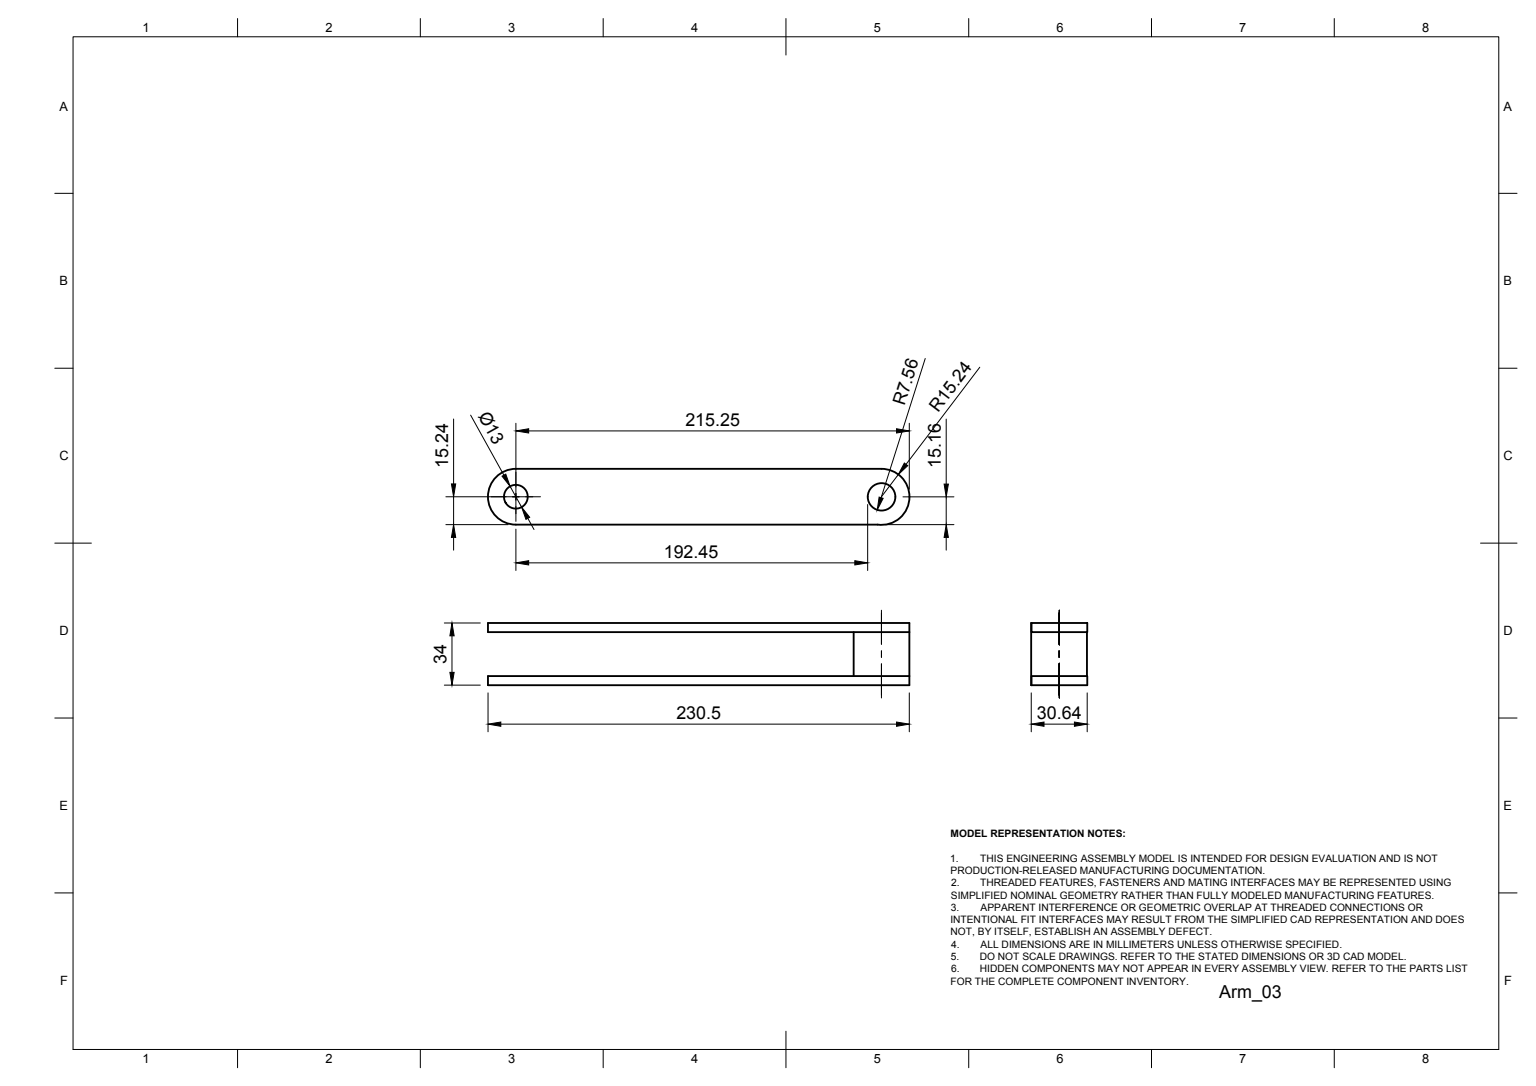
ISO-10303-21;
HEADER;
/* Generated by software containing ST-Developer
 * from STEP Tools, Inc. (www.steptools.com) 
 */

FILE_DESCRIPTION(
/* description */ (''),
/* implementation_level */ '2;1');

FILE_NAME(
/* name */ 'Arm_03.step',
/* time_stamp */ '2026-10-06T13:41:14-07:00',
/* author */ (''),
/* organization */ (''),
/* preprocessor_version */ 'ST-DEVELOPER v20.2',
/* originating_system */ 'Autodesk Translation Framework v15.15.0.0',
/* authorisation */ '');

FILE_SCHEMA (('AUTOMOTIVE_DESIGN { 1 0 10303 214 3 1 1 }'));
ENDSEC;

DATA;
#10=MECHANICAL_DESIGN_GEOMETRIC_PRESENTATION_REPRESENTATION('',(#1965),#279266);
#1947=SHAPE_REPRESENTATION_RELATIONSHIP('SRR','None',#279306,#1956);
#1956=ADVANCED_BREP_SHAPE_REPRESENTATION('',(#1974),#279262);
#1965=STYLED_ITEM('',(#279355),#1974);
#1974=MANIFOLD_SOLID_BREP('Body1',#14943);
#2002=FACE_BOUND('',#2985,.T.);
#2003=FACE_BOUND('',#2992,.T.);
#2004=FACE_BOUND('',#2993,.T.);
#2005=FACE_BOUND('',#2996,.T.);
#2006=FACE_BOUND('',#2997,.T.);
#2007=FACE_BOUND('',#2999,.T.);
#2071=PLANE('',#15521);
#2072=PLANE('',#15522);
#2073=PLANE('',#15526);
#2074=PLANE('',#15529);
#2075=PLANE('',#15534);
#2076=PLANE('',#15538);
#2077=PLANE('',#15542);
#2078=PLANE('',#15547);
#2079=PLANE('',#15549);
#2080=PLANE('',#15551);
#2486=FACE_OUTER_BOUND('',#2980,.T.);
#2487=FACE_OUTER_BOUND('',#2981,.T.);
#2488=FACE_OUTER_BOUND('',#2982,.T.);
#2489=FACE_OUTER_BOUND('',#2983,.T.);
#2490=FACE_OUTER_BOUND('',#2984,.T.);
#2491=FACE_OUTER_BOUND('',#2986,.T.);
#2492=FACE_OUTER_BOUND('',#2987,.T.);
#2493=FACE_OUTER_BOUND('',#2988,.T.);
#2494=FACE_OUTER_BOUND('',#2989,.T.);
#2495=FACE_OUTER_BOUND('',#2990,.T.);
#2496=FACE_OUTER_BOUND('',#2991,.T.);
#2497=FACE_OUTER_BOUND('',#2994,.T.);
#2498=FACE_OUTER_BOUND('',#2995,.T.);
#2499=FACE_OUTER_BOUND('',#2998,.T.);
#2500=FACE_OUTER_BOUND('',#3000,.T.);
#2501=FACE_OUTER_BOUND('',#3001,.T.);
#2502=FACE_OUTER_BOUND('',#3002,.T.);
#2503=FACE_OUTER_BOUND('',#3003,.T.);
#2504=FACE_OUTER_BOUND('',#3004,.T.);
#2505=FACE_OUTER_BOUND('',#3005,.T.);
#2980=EDGE_LOOP('',(#13442,#13443,#13444,#13445,#13446,#13447,#13448,#13449,
#13450,#13451,#13452,#13453));
#2981=EDGE_LOOP('',(#13454,#13455,#13456,#13457,#13458,#13459,#13460,#13461,
#13462,#13463,#13464,#13465));
#2982=EDGE_LOOP('',(#13466,#13467,#13468,#13469));
#2983=EDGE_LOOP('',(#13470,#13471,#13472,#13473));
#2984=EDGE_LOOP('',(#13474,#13475,#13476,#13477,#13478,#13479));
#2985=EDGE_LOOP('',(#13480));
#2986=EDGE_LOOP('',(#13481,#13482));
#2987=EDGE_LOOP('',(#13483,#13484,#13485,#13486));
#2988=EDGE_LOOP('',(#13487,#13488,#13489,#13490));
#2989=EDGE_LOOP('',(#13491,#13492,#13493,#13494));
#2990=EDGE_LOOP('',(#13495,#13496,#13497,#13498));
#2991=EDGE_LOOP('',(#13499,#13500,#13501,#13502,#13503));
#2992=EDGE_LOOP('',(#13504));
#2993=EDGE_LOOP('',(#13505,#13506,#13507));
#2994=EDGE_LOOP('',(#13508,#13509,#13510,#13511));
#2995=EDGE_LOOP('',(#13512,#13513,#13514,#13515,#13516));
#2996=EDGE_LOOP('',(#13517));
#2997=EDGE_LOOP('',(#13518,#13519,#13520));
#2998=EDGE_LOOP('',(#13521,#13522,#13523,#13524,#13525,#13526));
#2999=EDGE_LOOP('',(#13527));
#3000=EDGE_LOOP('',(#13528,#13529,#13530,#13531));
#3001=EDGE_LOOP('',(#13532,#13533,#13534,#13535));
#3002=EDGE_LOOP('',(#13536,#13537,#13538,#13539));
#3003=EDGE_LOOP('',(#13540,#13541,#13542,#13543));
#3004=EDGE_LOOP('',(#13544,#13545,#13546,#13547));
#3005=EDGE_LOOP('',(#13548,#13549));
#3499=LINE('',#240528,#4027);
#3500=LINE('',#240532,#4028);
#3501=LINE('',#240536,#4029);
#3502=LINE('',#240541,#4030);
#3503=LINE('',#240544,#4031);
#3504=LINE('',#240550,#4032);
#3505=LINE('',#240554,#4033);
#3506=LINE('',#240557,#4034);
#3507=LINE('',#240561,#4035);
#3508=LINE('',#240565,#4036);
#3509=LINE('',#240572,#4037);
#3510=LINE('',#240574,#4038);
#3511=LINE('',#240575,#4039);
#3512=LINE('',#240580,#4040);
#3513=LINE('',#240587,#4041);
#3514=LINE('',#240592,#4042);
#3515=LINE('',#240593,#4043);
#3516=LINE('',#240594,#4044);
#3517=LINE('',#240607,#4045);
#3518=LINE('',#240610,#4046);
#3519=LINE('',#240615,#4047);
#3520=LINE('',#240619,#4048);
#3521=LINE('',#240624,#4049);
#3522=LINE('',#240626,#4050);
#3523=LINE('',#240627,#4051);
#3524=LINE('',#240629,#4052);
#4027=VECTOR('',#16995,7.55784864301595);
#4028=VECTOR('',#16998,10.);
#4029=VECTOR('',#17001,10.);
#4030=VECTOR('',#17006,10.);
#4031=VECTOR('',#17009,10.);
#4032=VECTOR('',#17014,10.);
#4033=VECTOR('',#17017,10.);
#4034=VECTOR('',#17020,15.2420394990918);
#4035=VECTOR('',#17023,10.);
#4036=VECTOR('',#17026,10.);
#4037=VECTOR('',#17037,10.);
#4038=VECTOR('',#17038,10.);
#4039=VECTOR('',#17039,10.);
#4040=VECTOR('',#17044,10.);
#4041=VECTOR('',#17053,6.50110764916953);
#4042=VECTOR('',#17058,10.);
#4043=VECTOR('',#17059,10.);
#4044=VECTOR('',#17060,10.);
#4045=VECTOR('',#17081,10.);
#4046=VECTOR('',#17084,10.);
#4047=VECTOR('',#17089,10.);
#4048=VECTOR('',#17092,10.);
#4049=VECTOR('',#17099,6.50110764916953);
#4050=VECTOR('',#17102,10.);
#4051=VECTOR('',#17103,10.);
#4052=VECTOR('',#17106,10.);
#4232=CIRCLE('',#15505,7.55784864301595);
#4233=CIRCLE('',#15506,7.55784864301595);
#4234=CIRCLE('',#15507,7.55784864301595);
#4235=CIRCLE('',#15508,7.55784864301595);
#4236=CIRCLE('',#15509,7.55784864301595);
#4237=CIRCLE('',#15510,7.55784864301595);
#4238=CIRCLE('',#15512,15.2420394990918);
#4239=CIRCLE('',#15513,15.2420394990918);
#4240=CIRCLE('',#15514,15.2420394990918);
#4241=CIRCLE('',#15515,15.2420394990918);
#4242=CIRCLE('',#15516,15.2420394990918);
#4243=CIRCLE('',#15517,15.2420394990918);
#4244=CIRCLE('',#15519,7.55784864301595);
#4245=CIRCLE('',#15520,7.55784864301595);
#4246=CIRCLE('',#15523,15.2420394990918);
#4247=CIRCLE('',#15524,15.2420394990918);
#4248=CIRCLE('',#15525,6.50110764916953);
#4249=CIRCLE('',#15528,6.50110764916953);
#4250=CIRCLE('',#15531,15.2420394990918);
#4251=CIRCLE('',#15533,15.2420394990918);
#4252=CIRCLE('',#15536,7.55784864301595);
#4253=CIRCLE('',#15537,7.55784864301595);
#4254=CIRCLE('',#15539,15.2420394990918);
#4255=CIRCLE('',#15540,15.2420394990918);
#4256=CIRCLE('',#15541,6.50110764916953);
#4257=CIRCLE('',#15543,15.2420394990918);
#4258=CIRCLE('',#15544,15.2420394990918);
#4259=CIRCLE('',#15545,6.50110764916953);
#6171=VERTEX_POINT('',#240524);
#6172=VERTEX_POINT('',#240525);
#6173=VERTEX_POINT('',#240527);
#6174=VERTEX_POINT('',#240529);
#6175=VERTEX_POINT('',#240531);
#6176=VERTEX_POINT('',#240533);
#6177=VERTEX_POINT('',#240535);
#6178=VERTEX_POINT('',#240538);
#6179=VERTEX_POINT('',#240540);
#6180=VERTEX_POINT('',#240542);
#6181=VERTEX_POINT('',#240546);
#6182=VERTEX_POINT('',#240547);
#6183=VERTEX_POINT('',#240549);
#6184=VERTEX_POINT('',#240551);
#6185=VERTEX_POINT('',#240553);
#6186=VERTEX_POINT('',#240556);
#6187=VERTEX_POINT('',#240558);
#6188=VERTEX_POINT('',#240560);
#6189=VERTEX_POINT('',#240562);
#6190=VERTEX_POINT('',#240564);
#6191=VERTEX_POINT('',#240571);
#6192=VERTEX_POINT('',#240573);
#6193=VERTEX_POINT('',#240577);
#6194=VERTEX_POINT('',#240579);
#6195=VERTEX_POINT('',#240582);
#6196=VERTEX_POINT('',#240586);
#6197=VERTEX_POINT('',#240590);
#6198=VERTEX_POINT('',#240591);
#6199=VERTEX_POINT('',#240604);
#6200=VERTEX_POINT('',#240606);
#6201=VERTEX_POINT('',#240608);
#6202=VERTEX_POINT('',#240611);
#6203=VERTEX_POINT('',#240614);
#6204=VERTEX_POINT('',#240616);
#6205=VERTEX_POINT('',#240618);
#6206=VERTEX_POINT('',#240621);
#8646=EDGE_CURVE('',#6171,#6172,#4232,.T.);
#8647=EDGE_CURVE('',#6172,#6173,#3499,.T.);
#8648=EDGE_CURVE('',#6174,#6173,#4233,.T.);
#8649=EDGE_CURVE('',#6175,#6174,#3500,.T.);
#8650=EDGE_CURVE('',#6176,#6175,#4234,.T.);
#8651=EDGE_CURVE('',#6177,#6176,#3501,.T.);
#8652=EDGE_CURVE('',#6173,#6177,#4235,.T.);
#8653=EDGE_CURVE('',#6172,#6178,#4236,.T.);
#8654=EDGE_CURVE('',#6179,#6178,#3502,.T.);
#8655=EDGE_CURVE('',#6180,#6179,#4237,.T.);
#8656=EDGE_CURVE('',#6171,#6180,#3503,.T.);
#8657=EDGE_CURVE('',#6181,#6182,#4238,.T.);
#8658=EDGE_CURVE('',#6183,#6181,#3504,.T.);
#8659=EDGE_CURVE('',#6184,#6183,#4239,.T.);
#8660=EDGE_CURVE('',#6185,#6184,#3505,.T.);
#8661=EDGE_CURVE('',#6182,#6185,#4240,.T.);
#8662=EDGE_CURVE('',#6182,#6186,#3506,.T.);
#8663=EDGE_CURVE('',#6187,#6186,#4241,.T.);
#8664=EDGE_CURVE('',#6188,#6187,#3507,.T.);
#8665=EDGE_CURVE('',#6188,#6189,#4242,.T.);
#8666=EDGE_CURVE('',#6190,#6189,#3508,.T.);
#8667=EDGE_CURVE('',#6186,#6190,#4243,.T.);
#8668=EDGE_CURVE('',#6176,#6175,#4244,.T.);
#8669=EDGE_CURVE('',#6177,#6174,#4245,.T.);
#8670=EDGE_CURVE('',#6181,#6191,#3509,.T.);
#8671=EDGE_CURVE('',#6192,#6191,#3510,.T.);
#8672=EDGE_CURVE('',#6183,#6192,#3511,.T.);
#8673=EDGE_CURVE('',#6193,#6185,#4246,.T.);
#8674=EDGE_CURVE('',#6194,#6193,#3512,.T.);
#8675=EDGE_CURVE('',#6191,#6194,#4247,.T.);
#8676=EDGE_CURVE('',#6195,#6195,#4248,.T.);
#8677=EDGE_CURVE('',#6195,#6196,#3513,.T.);
#8678=EDGE_CURVE('',#6196,#6196,#4249,.T.);
#8679=EDGE_CURVE('',#6197,#6198,#3514,.T.);
#8680=EDGE_CURVE('',#6197,#6194,#3515,.T.);
#8681=EDGE_CURVE('',#6198,#6193,#3516,.T.);
#8682=EDGE_CURVE('',#6192,#6197,#4250,.T.);
#8683=EDGE_CURVE('',#6198,#6184,#4251,.T.);
#8684=EDGE_CURVE('',#6178,#6171,#4252,.T.);
#8685=EDGE_CURVE('',#6179,#6180,#4253,.T.);
#8686=EDGE_CURVE('',#6199,#6188,#4254,.T.);
#8687=EDGE_CURVE('',#6200,#6199,#3517,.T.);
#8688=EDGE_CURVE('',#6201,#6200,#4255,.T.);
#8689=EDGE_CURVE('',#6189,#6201,#3518,.T.);
#8690=EDGE_CURVE('',#6202,#6202,#4256,.T.);
#8691=EDGE_CURVE('',#6190,#6203,#3519,.T.);
#8692=EDGE_CURVE('',#6203,#6204,#4257,.T.);
#8693=EDGE_CURVE('',#6204,#6205,#3520,.T.);
#8694=EDGE_CURVE('',#6205,#6187,#4258,.T.);
#8695=EDGE_CURVE('',#6206,#6206,#4259,.T.);
#8696=EDGE_CURVE('',#6202,#6206,#3521,.T.);
#8697=EDGE_CURVE('',#6199,#6205,#3522,.T.);
#8698=EDGE_CURVE('',#6200,#6204,#3523,.T.);
#8699=EDGE_CURVE('',#6201,#6203,#3524,.T.);
#13442=ORIENTED_EDGE('',*,*,#8646,.T.);
#13443=ORIENTED_EDGE('',*,*,#8647,.T.);
#13444=ORIENTED_EDGE('',*,*,#8648,.F.);
#13445=ORIENTED_EDGE('',*,*,#8649,.F.);
#13446=ORIENTED_EDGE('',*,*,#8650,.F.);
#13447=ORIENTED_EDGE('',*,*,#8651,.F.);
#13448=ORIENTED_EDGE('',*,*,#8652,.F.);
#13449=ORIENTED_EDGE('',*,*,#8647,.F.);
#13450=ORIENTED_EDGE('',*,*,#8653,.T.);
#13451=ORIENTED_EDGE('',*,*,#8654,.F.);
#13452=ORIENTED_EDGE('',*,*,#8655,.F.);
#13453=ORIENTED_EDGE('',*,*,#8656,.F.);
#13454=ORIENTED_EDGE('',*,*,#8657,.F.);
#13455=ORIENTED_EDGE('',*,*,#8658,.F.);
#13456=ORIENTED_EDGE('',*,*,#8659,.F.);
#13457=ORIENTED_EDGE('',*,*,#8660,.F.);
#13458=ORIENTED_EDGE('',*,*,#8661,.F.);
#13459=ORIENTED_EDGE('',*,*,#8662,.T.);
#13460=ORIENTED_EDGE('',*,*,#8663,.F.);
#13461=ORIENTED_EDGE('',*,*,#8664,.F.);
#13462=ORIENTED_EDGE('',*,*,#8665,.T.);
#13463=ORIENTED_EDGE('',*,*,#8666,.F.);
#13464=ORIENTED_EDGE('',*,*,#8667,.F.);
#13465=ORIENTED_EDGE('',*,*,#8662,.F.);
#13466=ORIENTED_EDGE('',*,*,#8651,.T.);
#13467=ORIENTED_EDGE('',*,*,#8668,.T.);
#13468=ORIENTED_EDGE('',*,*,#8649,.T.);
#13469=ORIENTED_EDGE('',*,*,#8669,.F.);
#13470=ORIENTED_EDGE('',*,*,#8658,.T.);
#13471=ORIENTED_EDGE('',*,*,#8670,.T.);
#13472=ORIENTED_EDGE('',*,*,#8671,.F.);
#13473=ORIENTED_EDGE('',*,*,#8672,.F.);
#13474=ORIENTED_EDGE('',*,*,#8657,.T.);
#13475=ORIENTED_EDGE('',*,*,#8661,.T.);
#13476=ORIENTED_EDGE('',*,*,#8673,.F.);
#13477=ORIENTED_EDGE('',*,*,#8674,.F.);
#13478=ORIENTED_EDGE('',*,*,#8675,.F.);
#13479=ORIENTED_EDGE('',*,*,#8670,.F.);
#13480=ORIENTED_EDGE('',*,*,#8676,.F.);
#13481=ORIENTED_EDGE('',*,*,#8650,.T.);
#13482=ORIENTED_EDGE('',*,*,#8668,.F.);
#13483=ORIENTED_EDGE('',*,*,#8676,.T.);
#13484=ORIENTED_EDGE('',*,*,#8677,.T.);
#13485=ORIENTED_EDGE('',*,*,#8678,.F.);
#13486=ORIENTED_EDGE('',*,*,#8677,.F.);
#13487=ORIENTED_EDGE('',*,*,#8679,.F.);
#13488=ORIENTED_EDGE('',*,*,#8680,.T.);
#13489=ORIENTED_EDGE('',*,*,#8674,.T.);
#13490=ORIENTED_EDGE('',*,*,#8681,.F.);
#13491=ORIENTED_EDGE('',*,*,#8682,.F.);
#13492=ORIENTED_EDGE('',*,*,#8671,.T.);
#13493=ORIENTED_EDGE('',*,*,#8675,.T.);
#13494=ORIENTED_EDGE('',*,*,#8680,.F.);
#13495=ORIENTED_EDGE('',*,*,#8660,.T.);
#13496=ORIENTED_EDGE('',*,*,#8683,.F.);
#13497=ORIENTED_EDGE('',*,*,#8681,.T.);
#13498=ORIENTED_EDGE('',*,*,#8673,.T.);
#13499=ORIENTED_EDGE('',*,*,#8672,.T.);
#13500=ORIENTED_EDGE('',*,*,#8682,.T.);
#13501=ORIENTED_EDGE('',*,*,#8679,.T.);
#13502=ORIENTED_EDGE('',*,*,#8683,.T.);
#13503=ORIENTED_EDGE('',*,*,#8659,.T.);
#13504=ORIENTED_EDGE('',*,*,#8678,.T.);
#13505=ORIENTED_EDGE('',*,*,#8669,.T.);
#13506=ORIENTED_EDGE('',*,*,#8648,.T.);
#13507=ORIENTED_EDGE('',*,*,#8652,.T.);
#13508=ORIENTED_EDGE('',*,*,#8654,.T.);
#13509=ORIENTED_EDGE('',*,*,#8684,.T.);
#13510=ORIENTED_EDGE('',*,*,#8656,.T.);
#13511=ORIENTED_EDGE('',*,*,#8685,.F.);
#13512=ORIENTED_EDGE('',*,*,#8665,.F.);
#13513=ORIENTED_EDGE('',*,*,#8686,.F.);
#13514=ORIENTED_EDGE('',*,*,#8687,.F.);
#13515=ORIENTED_EDGE('',*,*,#8688,.F.);
#13516=ORIENTED_EDGE('',*,*,#8689,.F.);
#13517=ORIENTED_EDGE('',*,*,#8690,.F.);
#13518=ORIENTED_EDGE('',*,*,#8684,.F.);
#13519=ORIENTED_EDGE('',*,*,#8653,.F.);
#13520=ORIENTED_EDGE('',*,*,#8646,.F.);
#13521=ORIENTED_EDGE('',*,*,#8663,.T.);
#13522=ORIENTED_EDGE('',*,*,#8667,.T.);
#13523=ORIENTED_EDGE('',*,*,#8691,.T.);
#13524=ORIENTED_EDGE('',*,*,#8692,.T.);
#13525=ORIENTED_EDGE('',*,*,#8693,.T.);
#13526=ORIENTED_EDGE('',*,*,#8694,.T.);
#13527=ORIENTED_EDGE('',*,*,#8695,.T.);
#13528=ORIENTED_EDGE('',*,*,#8690,.T.);
#13529=ORIENTED_EDGE('',*,*,#8696,.T.);
#13530=ORIENTED_EDGE('',*,*,#8695,.F.);
#13531=ORIENTED_EDGE('',*,*,#8696,.F.);
#13532=ORIENTED_EDGE('',*,*,#8687,.T.);
#13533=ORIENTED_EDGE('',*,*,#8697,.T.);
#13534=ORIENTED_EDGE('',*,*,#8693,.F.);
#13535=ORIENTED_EDGE('',*,*,#8698,.F.);
#13536=ORIENTED_EDGE('',*,*,#8688,.T.);
#13537=ORIENTED_EDGE('',*,*,#8698,.T.);
#13538=ORIENTED_EDGE('',*,*,#8692,.F.);
#13539=ORIENTED_EDGE('',*,*,#8699,.F.);
#13540=ORIENTED_EDGE('',*,*,#8666,.T.);
#13541=ORIENTED_EDGE('',*,*,#8689,.T.);
#13542=ORIENTED_EDGE('',*,*,#8699,.T.);
#13543=ORIENTED_EDGE('',*,*,#8691,.F.);
#13544=ORIENTED_EDGE('',*,*,#8664,.T.);
#13545=ORIENTED_EDGE('',*,*,#8694,.F.);
#13546=ORIENTED_EDGE('',*,*,#8697,.F.);
#13547=ORIENTED_EDGE('',*,*,#8686,.T.);
#13548=ORIENTED_EDGE('',*,*,#8655,.T.);
#13549=ORIENTED_EDGE('',*,*,#8685,.T.);
#14417=CYLINDRICAL_SURFACE('',#15504,7.55784864301595);
#14418=CYLINDRICAL_SURFACE('',#15511,15.2420394990918);
#14419=CYLINDRICAL_SURFACE('',#15518,7.55784864301595);
#14420=CYLINDRICAL_SURFACE('',#15527,6.50110764916953);
#14421=CYLINDRICAL_SURFACE('',#15530,15.2420394990918);
#14422=CYLINDRICAL_SURFACE('',#15532,15.2420394990918);
#14423=CYLINDRICAL_SURFACE('',#15535,7.55784864301595);
#14424=CYLINDRICAL_SURFACE('',#15546,6.50110764916953);
#14425=CYLINDRICAL_SURFACE('',#15548,15.2420394990918);
#14426=CYLINDRICAL_SURFACE('',#15550,15.2420394990918);
#14844=ADVANCED_FACE('',(#2486),#14417,.F.);
#14845=ADVANCED_FACE('',(#2487),#14418,.T.);
#14846=ADVANCED_FACE('',(#2488),#14419,.F.);
#14847=ADVANCED_FACE('',(#2489),#2071,.F.);
#14848=ADVANCED_FACE('',(#2490,#2002),#2072,.F.);
#14849=ADVANCED_FACE('',(#2491),#2073,.F.);
#14850=ADVANCED_FACE('',(#2492),#14420,.F.);
#14851=ADVANCED_FACE('',(#2493),#2074,.F.);
#14852=ADVANCED_FACE('',(#2494),#14421,.T.);
#14853=ADVANCED_FACE('',(#2495),#14422,.T.);
#14854=ADVANCED_FACE('',(#2496,#2003,#2004),#2075,.T.);
#14855=ADVANCED_FACE('',(#2497),#14423,.F.);
#14856=ADVANCED_FACE('',(#2498,#2005,#2006),#2076,.F.);
#14857=ADVANCED_FACE('',(#2499,#2007),#2077,.T.);
#14858=ADVANCED_FACE('',(#2500),#14424,.F.);
#14859=ADVANCED_FACE('',(#2501),#2078,.T.);
#14860=ADVANCED_FACE('',(#2502),#14425,.T.);
#14861=ADVANCED_FACE('',(#2503),#2079,.T.);
#14862=ADVANCED_FACE('',(#2504),#14426,.T.);
#14863=ADVANCED_FACE('',(#2505),#2080,.T.);
#14943=CLOSED_SHELL('',(#14844,#14845,#14846,#14847,#14848,#14849,#14850,
#14851,#14852,#14853,#14854,#14855,#14856,#14857,#14858,#14859,#14860,#14861,
#14862,#14863));
#15503=AXIS2_PLACEMENT_3D('',#240522,#16989,#16990);
#15504=AXIS2_PLACEMENT_3D('',#240523,#16991,#16992);
#15505=AXIS2_PLACEMENT_3D('',#240526,#16993,#16994);
#15506=AXIS2_PLACEMENT_3D('',#240530,#16996,#16997);
#15507=AXIS2_PLACEMENT_3D('',#240534,#16999,#17000);
#15508=AXIS2_PLACEMENT_3D('',#240537,#17002,#17003);
#15509=AXIS2_PLACEMENT_3D('',#240539,#17004,#17005);
#15510=AXIS2_PLACEMENT_3D('',#240543,#17007,#17008);
#15511=AXIS2_PLACEMENT_3D('',#240545,#17010,#17011);
#15512=AXIS2_PLACEMENT_3D('',#240548,#17012,#17013);
#15513=AXIS2_PLACEMENT_3D('',#240552,#17015,#17016);
#15514=AXIS2_PLACEMENT_3D('',#240555,#17018,#17019);
#15515=AXIS2_PLACEMENT_3D('',#240559,#17021,#17022);
#15516=AXIS2_PLACEMENT_3D('',#240563,#17024,#17025);
#15517=AXIS2_PLACEMENT_3D('',#240566,#17027,#17028);
#15518=AXIS2_PLACEMENT_3D('',#240567,#17029,#17030);
#15519=AXIS2_PLACEMENT_3D('',#240568,#17031,#17032);
#15520=AXIS2_PLACEMENT_3D('',#240569,#17033,#17034);
#15521=AXIS2_PLACEMENT_3D('',#240570,#17035,#17036);
#15522=AXIS2_PLACEMENT_3D('',#240576,#17040,#17041);
#15523=AXIS2_PLACEMENT_3D('',#240578,#17042,#17043);
#15524=AXIS2_PLACEMENT_3D('',#240581,#17045,#17046);
#15525=AXIS2_PLACEMENT_3D('',#240583,#17047,#17048);
#15526=AXIS2_PLACEMENT_3D('',#240584,#17049,#17050);
#15527=AXIS2_PLACEMENT_3D('',#240585,#17051,#17052);
#15528=AXIS2_PLACEMENT_3D('',#240588,#17054,#17055);
#15529=AXIS2_PLACEMENT_3D('',#240589,#17056,#17057);
#15530=AXIS2_PLACEMENT_3D('',#240595,#17061,#17062);
#15531=AXIS2_PLACEMENT_3D('',#240596,#17063,#17064);
#15532=AXIS2_PLACEMENT_3D('',#240597,#17065,#17066);
#15533=AXIS2_PLACEMENT_3D('',#240598,#17067,#17068);
#15534=AXIS2_PLACEMENT_3D('',#240599,#17069,#17070);
#15535=AXIS2_PLACEMENT_3D('',#240600,#17071,#17072);
#15536=AXIS2_PLACEMENT_3D('',#240601,#17073,#17074);
#15537=AXIS2_PLACEMENT_3D('',#240602,#17075,#17076);
#15538=AXIS2_PLACEMENT_3D('',#240603,#17077,#17078);
#15539=AXIS2_PLACEMENT_3D('',#240605,#17079,#17080);
#15540=AXIS2_PLACEMENT_3D('',#240609,#17082,#17083);
#15541=AXIS2_PLACEMENT_3D('',#240612,#17085,#17086);
#15542=AXIS2_PLACEMENT_3D('',#240613,#17087,#17088);
#15543=AXIS2_PLACEMENT_3D('',#240617,#17090,#17091);
#15544=AXIS2_PLACEMENT_3D('',#240620,#17093,#17094);
#15545=AXIS2_PLACEMENT_3D('',#240622,#17095,#17096);
#15546=AXIS2_PLACEMENT_3D('',#240623,#17097,#17098);
#15547=AXIS2_PLACEMENT_3D('',#240625,#17100,#17101);
#15548=AXIS2_PLACEMENT_3D('',#240628,#17104,#17105);
#15549=AXIS2_PLACEMENT_3D('',#240630,#17107,#17108);
#15550=AXIS2_PLACEMENT_3D('',#240631,#17109,#17110);
#15551=AXIS2_PLACEMENT_3D('',#240632,#17111,#17112);
#16989=DIRECTION('axis',(0.,0.,1.));
#16990=DIRECTION('refdir',(1.,0.,0.));
#16991=DIRECTION('center_axis',(0.,1.,0.));
#16992=DIRECTION('ref_axis',(1.,0.,0.));
#16993=DIRECTION('center_axis',(0.,-1.,0.));
#16994=DIRECTION('ref_axis',(1.,0.,0.));
#16995=DIRECTION('',(0.,1.,0.));
#16996=DIRECTION('center_axis',(0.,-1.,0.));
#16997=DIRECTION('ref_axis',(1.,0.,0.));
#16998=DIRECTION('',(0.,1.,0.));
#16999=DIRECTION('center_axis',(0.,-1.,0.));
#17000=DIRECTION('ref_axis',(1.,0.,0.));
#17001=DIRECTION('',(0.,-1.,0.));
#17002=DIRECTION('center_axis',(0.,-1.,0.));
#17003=DIRECTION('ref_axis',(1.,0.,0.));
#17004=DIRECTION('center_axis',(0.,-1.,0.));
#17005=DIRECTION('ref_axis',(1.,0.,0.));
#17006=DIRECTION('',(0.,-1.,0.));
#17007=DIRECTION('center_axis',(0.,1.,0.));
#17008=DIRECTION('ref_axis',(1.,0.,0.));
#17009=DIRECTION('',(0.,1.,0.));
#17010=DIRECTION('center_axis',(0.,1.,0.));
#17011=DIRECTION('ref_axis',(1.,0.,0.));
#17012=DIRECTION('center_axis',(0.,1.,0.));
#17013=DIRECTION('ref_axis',(1.,0.,0.));
#17014=DIRECTION('',(0.,-1.,0.));
#17015=DIRECTION('center_axis',(0.,1.,0.));
#17016=DIRECTION('ref_axis',(1.,0.,0.));
#17017=DIRECTION('',(0.,1.,0.));
#17018=DIRECTION('center_axis',(0.,1.,0.));
#17019=DIRECTION('ref_axis',(1.,0.,0.));
#17020=DIRECTION('',(0.,-1.,0.));
#17021=DIRECTION('center_axis',(0.,-1.,0.));
#17022=DIRECTION('ref_axis',(1.,0.,0.));
#17023=DIRECTION('',(0.,1.,0.));
#17024=DIRECTION('center_axis',(0.,1.,0.));
#17025=DIRECTION('ref_axis',(1.,0.,0.));
#17026=DIRECTION('',(0.,-1.,0.));
#17027=DIRECTION('center_axis',(0.,-1.,0.));
#17028=DIRECTION('ref_axis',(1.,0.,0.));
#17029=DIRECTION('center_axis',(0.,1.,0.));
#17030=DIRECTION('ref_axis',(0.503773977045354,0.,0.863835505204496));
#17031=DIRECTION('center_axis',(-1.19937668507924E-53,-1.,2.1198911140988E-53));
#17032=DIRECTION('ref_axis',(0.492423560103467,-2.43566064310008E-53,-0.8703556959399));
#17033=DIRECTION('center_axis',(-1.19937668507924E-53,-1.,2.1198911140988E-53));
#17034=DIRECTION('ref_axis',(0.492423560103467,-2.43566064310008E-53,-0.8703556959399));
#17035=DIRECTION('center_axis',(-0.503443599526487,0.,-0.864028091033974));
#17036=DIRECTION('ref_axis',(0.864028091033974,0.,-0.503443599526487));
#17037=DIRECTION('',(0.864028091033974,0.,-0.503443599526487));
#17038=DIRECTION('',(0.,-1.,0.));
#17039=DIRECTION('',(0.864028091033974,0.,-0.503443599526487));
#17040=DIRECTION('center_axis',(0.,1.,0.));
#17041=DIRECTION('ref_axis',(0.492423560103467,0.,-0.8703556959399));
#17042=DIRECTION('center_axis',(0.,1.,0.));
#17043=DIRECTION('ref_axis',(-0.503443599526488,0.,-0.864028091033974));
#17044=DIRECTION('',(-0.864028091033974,0.,0.503443599526487));
#17045=DIRECTION('center_axis',(0.,1.,0.));
#17046=DIRECTION('ref_axis',(0.503443599526489,0.,0.864028091033974));
#17047=DIRECTION('center_axis',(0.,-1.,0.));
#17048=DIRECTION('ref_axis',(0.492423560103467,0.,-0.8703556959399));
#17049=DIRECTION('center_axis',(0.,1.,0.));
#17050=DIRECTION('ref_axis',(0.492423560103467,0.,-0.8703556959399));
#17051=DIRECTION('center_axis',(0.,1.,0.));
#17052=DIRECTION('ref_axis',(0.492423560103467,0.,-0.8703556959399));
#17053=DIRECTION('',(0.,1.,0.));
#17054=DIRECTION('center_axis',(0.,-1.,0.));
#17055=DIRECTION('ref_axis',(0.492423560103467,0.,-0.8703556959399));
#17056=DIRECTION('center_axis',(0.503443599526487,0.,0.864028091033974));
#17057=DIRECTION('ref_axis',(-0.864028091033974,0.,0.503443599526487));
#17058=DIRECTION('',(-0.864028091033974,0.,0.503443599526487));
#17059=DIRECTION('',(0.,-1.,0.));
#17060=DIRECTION('',(0.,-1.,0.));
#17061=DIRECTION('center_axis',(0.,1.,0.));
#17062=DIRECTION('ref_axis',(0.503443599526489,0.,0.864028091033974));
#17063=DIRECTION('center_axis',(0.,1.,0.));
#17064=DIRECTION('ref_axis',(0.503443599526489,0.,0.864028091033974));
#17065=DIRECTION('center_axis',(0.,1.,0.));
#17066=DIRECTION('ref_axis',(-0.503443599526488,0.,-0.864028091033974));
#17067=DIRECTION('center_axis',(0.,1.,0.));
#17068=DIRECTION('ref_axis',(-0.503443599526488,0.,-0.864028091033974));
#17069=DIRECTION('center_axis',(0.,1.,0.));
#17070=DIRECTION('ref_axis',(0.492423560103467,0.,-0.8703556959399));
#17071=DIRECTION('center_axis',(0.,1.,0.));
#17072=DIRECTION('ref_axis',(0.503773977045354,0.,0.863835505204496));
#17073=DIRECTION('center_axis',(1.19937668507924E-53,-1.,-2.1198911140988E-53));
#17074=DIRECTION('ref_axis',(0.492423560103467,2.43566064310008E-53,-0.8703556959399));
#17075=DIRECTION('center_axis',(1.19937668507924E-53,-1.,-2.1198911140988E-53));
#17076=DIRECTION('ref_axis',(0.492423560103467,2.43566064310008E-53,-0.8703556959399));
#17077=DIRECTION('center_axis',(0.,1.,0.));
#17078=DIRECTION('ref_axis',(0.492423560103467,0.,-0.8703556959399));
#17079=DIRECTION('center_axis',(0.,1.,0.));
#17080=DIRECTION('ref_axis',(-0.503443599526488,0.,-0.864028091033974));
#17081=DIRECTION('',(-0.864028091033974,0.,0.503443599526487));
#17082=DIRECTION('center_axis',(0.,1.,0.));
#17083=DIRECTION('ref_axis',(0.503443599526489,0.,0.864028091033974));
#17084=DIRECTION('',(0.864028091033974,0.,-0.503443599526487));
#17085=DIRECTION('center_axis',(0.,-1.,0.));
#17086=DIRECTION('ref_axis',(0.492423560103467,0.,-0.8703556959399));
#17087=DIRECTION('center_axis',(0.,1.,0.));
#17088=DIRECTION('ref_axis',(0.492423560103467,0.,-0.8703556959399));
#17089=DIRECTION('',(0.864028091033974,0.,-0.503443599526487));
#17090=DIRECTION('center_axis',(0.,1.,0.));
#17091=DIRECTION('ref_axis',(0.503443599526489,0.,0.864028091033974));
#17092=DIRECTION('',(-0.864028091033974,0.,0.503443599526487));
#17093=DIRECTION('center_axis',(0.,1.,0.));
#17094=DIRECTION('ref_axis',(-0.503443599526488,0.,-0.864028091033974));
#17095=DIRECTION('center_axis',(0.,-1.,0.));
#17096=DIRECTION('ref_axis',(0.492423560103467,0.,-0.8703556959399));
#17097=DIRECTION('center_axis',(0.,1.,0.));
#17098=DIRECTION('ref_axis',(0.492423560103467,0.,-0.8703556959399));
#17099=DIRECTION('',(0.,1.,0.));
#17100=DIRECTION('center_axis',(-0.503443599526487,0.,-0.864028091033974));
#17101=DIRECTION('ref_axis',(-0.864028091033974,0.,0.503443599526487));
#17102=DIRECTION('',(0.,1.,0.));
#17103=DIRECTION('',(0.,1.,0.));
#17104=DIRECTION('center_axis',(0.,1.,0.));
#17105=DIRECTION('ref_axis',(0.503443599526489,0.,0.864028091033974));
#17106=DIRECTION('',(0.,1.,0.));
#17107=DIRECTION('center_axis',(0.503443599526487,0.,0.864028091033974));
#17108=DIRECTION('ref_axis',(0.864028091033974,0.,-0.503443599526487));
#17109=DIRECTION('center_axis',(0.,1.,0.));
#17110=DIRECTION('ref_axis',(-0.503443599526488,0.,-0.864028091033974));
#17111=DIRECTION('center_axis',(0.,1.,0.));
#17112=DIRECTION('ref_axis',(0.492423560103467,0.,-0.8703556959399));
#240522=CARTESIAN_POINT('',(0.,0.,0.));
#240523=CARTESIAN_POINT('Origin',(19.9792411332937,17.,231.631408332131));
#240524=CARTESIAN_POINT('',(13.4123053085775,-17.,235.37258862514));
#240525=CARTESIAN_POINT('',(12.4213924902778,-17.,231.631408332131));
#240526=CARTESIAN_POINT('Origin',(19.9792411332937,-17.,231.631408332131));
#240527=CARTESIAN_POINT('',(12.4213924902778,17.,231.631408332131));
#240528=CARTESIAN_POINT('',(12.4213924902778,17.,231.631408332131));
#240529=CARTESIAN_POINT('',(13.4123053085775,17.,235.37258862514));
#240530=CARTESIAN_POINT('Origin',(19.9792411332937,17.,231.631408332131));
#240531=CARTESIAN_POINT('',(13.4123053085775,12.,235.37258862514));
#240532=CARTESIAN_POINT('',(13.4123053085775,17.,235.37258862514));
#240533=CARTESIAN_POINT('',(26.4691126286313,12.,227.758083651093));
#240534=CARTESIAN_POINT('Origin',(19.9792411332937,12.,231.631408332131));
#240535=CARTESIAN_POINT('',(26.4691126286313,17.,227.758083651093));
#240536=CARTESIAN_POINT('',(26.4691126286313,17.,227.758083651093));
#240537=CARTESIAN_POINT('Origin',(19.9792411332937,17.,231.631408332131));
#240538=CARTESIAN_POINT('',(26.4691126286313,-17.,227.758083651093));
#240539=CARTESIAN_POINT('Origin',(19.9792411332937,-17.,231.631408332131));
#240540=CARTESIAN_POINT('',(26.4691126286313,-12.,227.758083651093));
#240541=CARTESIAN_POINT('',(26.4691126286313,17.,227.758083651093));
#240542=CARTESIAN_POINT('',(13.4123053085775,-12.,235.37258862514));
#240543=CARTESIAN_POINT('Origin',(19.9792411332937,-12.,231.631408332131));
#240544=CARTESIAN_POINT('',(13.4123053085775,17.,235.37258862514));
#240545=CARTESIAN_POINT('Origin',(19.9792411332937,17.,231.631408332131));
#240546=CARTESIAN_POINT('',(29.4368821049519,12.,243.584349198005));
#240547=CARTESIAN_POINT('',(4.7372016342019,12.,231.631408332131));
#240548=CARTESIAN_POINT('Origin',(19.9792411332937,12.,231.631408332131));
#240549=CARTESIAN_POINT('',(29.4368821049519,17.,243.584349198005));
#240550=CARTESIAN_POINT('',(29.4368821049519,17.,243.584349198005));
#240551=CARTESIAN_POINT('',(6.77425985905829,17.,239.243782313943));
#240552=CARTESIAN_POINT('Origin',(19.9792411332937,17.,231.631408332131));
#240553=CARTESIAN_POINT('',(6.77425985905829,12.,239.243782313943));
#240554=CARTESIAN_POINT('',(6.77425985905829,17.,239.243782313943));
#240555=CARTESIAN_POINT('Origin',(19.9792411332937,12.,231.631408332131));
#240556=CARTESIAN_POINT('',(4.7372016342019,-12.,231.631408332131));
#240557=CARTESIAN_POINT('',(4.7372016342019,17.,231.631408332131));
#240558=CARTESIAN_POINT('',(6.77425985905829,-12.,239.243782313943));
#240559=CARTESIAN_POINT('Origin',(19.9792411332937,-12.,231.631408332131));
#240560=CARTESIAN_POINT('',(6.77425985905829,-17.,239.243782313943));
#240561=CARTESIAN_POINT('',(6.77425985905829,17.,239.243782313943));
#240562=CARTESIAN_POINT('',(29.4368821049519,-17.,243.584349198005));
#240563=CARTESIAN_POINT('Origin',(19.9792411332937,-17.,231.631408332131));
#240564=CARTESIAN_POINT('',(29.4368821049519,-12.,243.584349198005));
#240565=CARTESIAN_POINT('',(29.4368821049519,17.,243.584349198005));
#240566=CARTESIAN_POINT('Origin',(19.9792411332937,-12.,231.631408332131));
#240567=CARTESIAN_POINT('Origin',(19.9021768039151,17.,231.499263944101));
#240568=CARTESIAN_POINT('Origin',(19.9021768039151,12.,231.499263944101));
#240569=CARTESIAN_POINT('Origin',(19.9021768039151,17.,231.499263944101));
#240570=CARTESIAN_POINT('Origin',(27.5756840334628,17.,244.668814235966));
#240571=CARTESIAN_POINT('',(200.391914451146,12.,143.97391090943));
#240572=CARTESIAN_POINT('',(27.5756840334628,12.,244.668814235966));
#240573=CARTESIAN_POINT('',(200.391914451146,17.,143.97391090943));
#240574=CARTESIAN_POINT('',(200.391914451146,17.,143.97391090943));
#240575=CARTESIAN_POINT('',(27.5756840334628,17.,244.668814235966));
#240576=CARTESIAN_POINT('Origin',(106.310292012757,12.,181.151812280833));
#240577=CARTESIAN_POINT('',(12.2286695743674,12.,218.329713652237));
#240578=CARTESIAN_POINT('Origin',(19.9021768039151,12.,231.499263944101));
#240579=CARTESIAN_POINT('',(185.044899992051,12.,117.634810325701));
#240580=CARTESIAN_POINT('',(185.044899992051,12.,117.634810325701));
#240581=CARTESIAN_POINT('Origin',(192.718407221598,12.,130.804360617566));
#240582=CARTESIAN_POINT('',(189.517108648379,12.,136.462636689939));
#240583=CARTESIAN_POINT('Origin',(192.718407221598,12.,130.804360617566));
#240584=CARTESIAN_POINT('Origin',(106.310292012757,12.,181.151812280833));
#240585=CARTESIAN_POINT('Origin',(192.718407221598,17.,130.804360617566));
#240586=CARTESIAN_POINT('',(189.517108648379,17.,136.462636689939));
#240587=CARTESIAN_POINT('',(189.517108648378,17.,136.462636689939));
#240588=CARTESIAN_POINT('Origin',(192.718407221598,17.,130.804360617566));
#240589=CARTESIAN_POINT('Origin',(185.044899992051,17.,117.634810325701));
#240590=CARTESIAN_POINT('',(185.044899992051,17.,117.634810325701));
#240591=CARTESIAN_POINT('',(12.2286695743674,17.,218.329713652237));
#240592=CARTESIAN_POINT('',(185.044899992051,17.,117.634810325701));
#240593=CARTESIAN_POINT('',(185.044899992051,17.,117.634810325701));
#240594=CARTESIAN_POINT('',(12.2286695743674,17.,218.329713652237));
#240595=CARTESIAN_POINT('Origin',(192.718407221598,17.,130.804360617566));
#240596=CARTESIAN_POINT('Origin',(192.718407221598,17.,130.804360617566));
#240597=CARTESIAN_POINT('Origin',(19.9021768039151,17.,231.499263944101));
#240598=CARTESIAN_POINT('Origin',(19.9021768039151,17.,231.499263944101));
#240599=CARTESIAN_POINT('Origin',(106.310292012757,17.,181.151812280833));
#240600=CARTESIAN_POINT('Origin',(19.9021768039151,-17.,231.499263944101));
#240601=CARTESIAN_POINT('Origin',(19.9021768039151,-17.,231.499263944101));
#240602=CARTESIAN_POINT('Origin',(19.9021768039151,-12.,231.499263944101));
#240603=CARTESIAN_POINT('Origin',(106.310292012757,-17.,181.151812280833));
#240604=CARTESIAN_POINT('',(12.2286695743674,-17.,218.329713652237));
#240605=CARTESIAN_POINT('Origin',(19.9021768039151,-17.,231.499263944101));
#240606=CARTESIAN_POINT('',(185.044899992051,-17.,117.634810325701));
#240607=CARTESIAN_POINT('',(185.044899992051,-17.,117.634810325701));
#240608=CARTESIAN_POINT('',(200.391914451146,-17.,143.97391090943));
#240609=CARTESIAN_POINT('Origin',(192.718407221598,-17.,130.804360617566));
#240610=CARTESIAN_POINT('',(27.5756840334628,-17.,244.668814235966));
#240611=CARTESIAN_POINT('',(189.517108648379,-17.,136.462636689939));
#240612=CARTESIAN_POINT('Origin',(192.718407221598,-17.,130.804360617566));
#240613=CARTESIAN_POINT('Origin',(106.310292012757,-12.,181.151812280833));
#240614=CARTESIAN_POINT('',(200.391914451146,-12.,143.97391090943));
#240615=CARTESIAN_POINT('',(27.5756840334628,-12.,244.668814235966));
#240616=CARTESIAN_POINT('',(185.044899992051,-12.,117.634810325701));
#240617=CARTESIAN_POINT('Origin',(192.718407221598,-12.,130.804360617566));
#240618=CARTESIAN_POINT('',(12.2286695743674,-12.,218.329713652237));
#240619=CARTESIAN_POINT('',(185.044899992051,-12.,117.634810325701));
#240620=CARTESIAN_POINT('Origin',(19.9021768039151,-12.,231.499263944101));
#240621=CARTESIAN_POINT('',(189.517108648379,-12.,136.462636689939));
#240622=CARTESIAN_POINT('Origin',(192.718407221598,-12.,130.804360617566));
#240623=CARTESIAN_POINT('Origin',(192.718407221598,-17.,130.804360617566));
#240624=CARTESIAN_POINT('',(189.517108648378,-17.,136.462636689939));
#240625=CARTESIAN_POINT('Origin',(185.044899992051,-17.,117.634810325701));
#240626=CARTESIAN_POINT('',(12.2286695743674,-17.,218.329713652237));
#240627=CARTESIAN_POINT('',(185.044899992051,-17.,117.634810325701));
#240628=CARTESIAN_POINT('Origin',(192.718407221598,-17.,130.804360617566));
#240629=CARTESIAN_POINT('',(200.391914451146,-17.,143.97391090943));
#240630=CARTESIAN_POINT('Origin',(27.5756840334628,-17.,244.668814235966));
#240631=CARTESIAN_POINT('Origin',(19.9021768039151,-17.,231.499263944101));
#240632=CARTESIAN_POINT('Origin',(106.310292012757,-12.,181.151812280833));
#279251=UNCERTAINTY_MEASURE_WITH_UNIT(LENGTH_MEASURE(0.01),#279267,
'DISTANCE_ACCURACY_VALUE',
'Maximum model space distance between geometric entities at asserted c
onnectivities');
#279255=UNCERTAINTY_MEASURE_WITH_UNIT(LENGTH_MEASURE(0.01),#279267,
'DISTANCE_ACCURACY_VALUE',
'Maximum model space distance between geometric entities at asserted c
onnectivities');
#279262=(
GEOMETRIC_REPRESENTATION_CONTEXT(3)
GLOBAL_UNCERTAINTY_ASSIGNED_CONTEXT((#279251))
GLOBAL_UNIT_ASSIGNED_CONTEXT((#279267,#279269,#279270))
REPRESENTATION_CONTEXT('','3D')
);
#279266=(
GEOMETRIC_REPRESENTATION_CONTEXT(3)
GLOBAL_UNCERTAINTY_ASSIGNED_CONTEXT((#279255))
GLOBAL_UNIT_ASSIGNED_CONTEXT((#279267,#279269,#279270))
REPRESENTATION_CONTEXT('','3D')
);
#279267=(
LENGTH_UNIT()
NAMED_UNIT(*)
SI_UNIT(.MILLI.,.METRE.)
);
#279269=(
NAMED_UNIT(*)
PLANE_ANGLE_UNIT()
SI_UNIT($,.RADIAN.)
);
#279270=(
NAMED_UNIT(*)
SI_UNIT($,.STERADIAN.)
SOLID_ANGLE_UNIT()
);
#279277=SHAPE_DEFINITION_REPRESENTATION(#279287,#279306);
#279287=PRODUCT_DEFINITION_SHAPE('',$,#279317);
#279306=SHAPE_REPRESENTATION('',(#15503),#279262);
#279310=PRODUCT_DEFINITION_CONTEXT('part definition',#279342,'design');
#279317=PRODUCT_DEFINITION('Arm_03','Arm_03',#279327,#279310);
#279327=PRODUCT_DEFINITION_FORMATION('',$,#279350);
#279342=APPLICATION_CONTEXT(
'Core Data for Automotive Mechanical Design Process');
#279343=PRODUCT_CONTEXT('part definition',#279342,'mechanical');
#279350=PRODUCT('Arm_03','Arm_03',$,(#279343));
#279355=PRESENTATION_STYLE_ASSIGNMENT((#279357));
#279357=SURFACE_STYLE_USAGE(.BOTH.,#279359);
#279359=SURFACE_SIDE_STYLE('',(#279361));
#279361=SURFACE_STYLE_FILL_AREA(#279363);
#279363=FILL_AREA_STYLE('Opaque(160,160,160)',(#279365));
#279365=FILL_AREA_STYLE_COLOUR('Opaque(160,160,160)',#279367);
#279367=COLOUR_RGB('Opaque(160,160,160)', 0.66274510, 0.83137255, 0.94901961);
ENDSEC;
END-ISO-10303-21;
